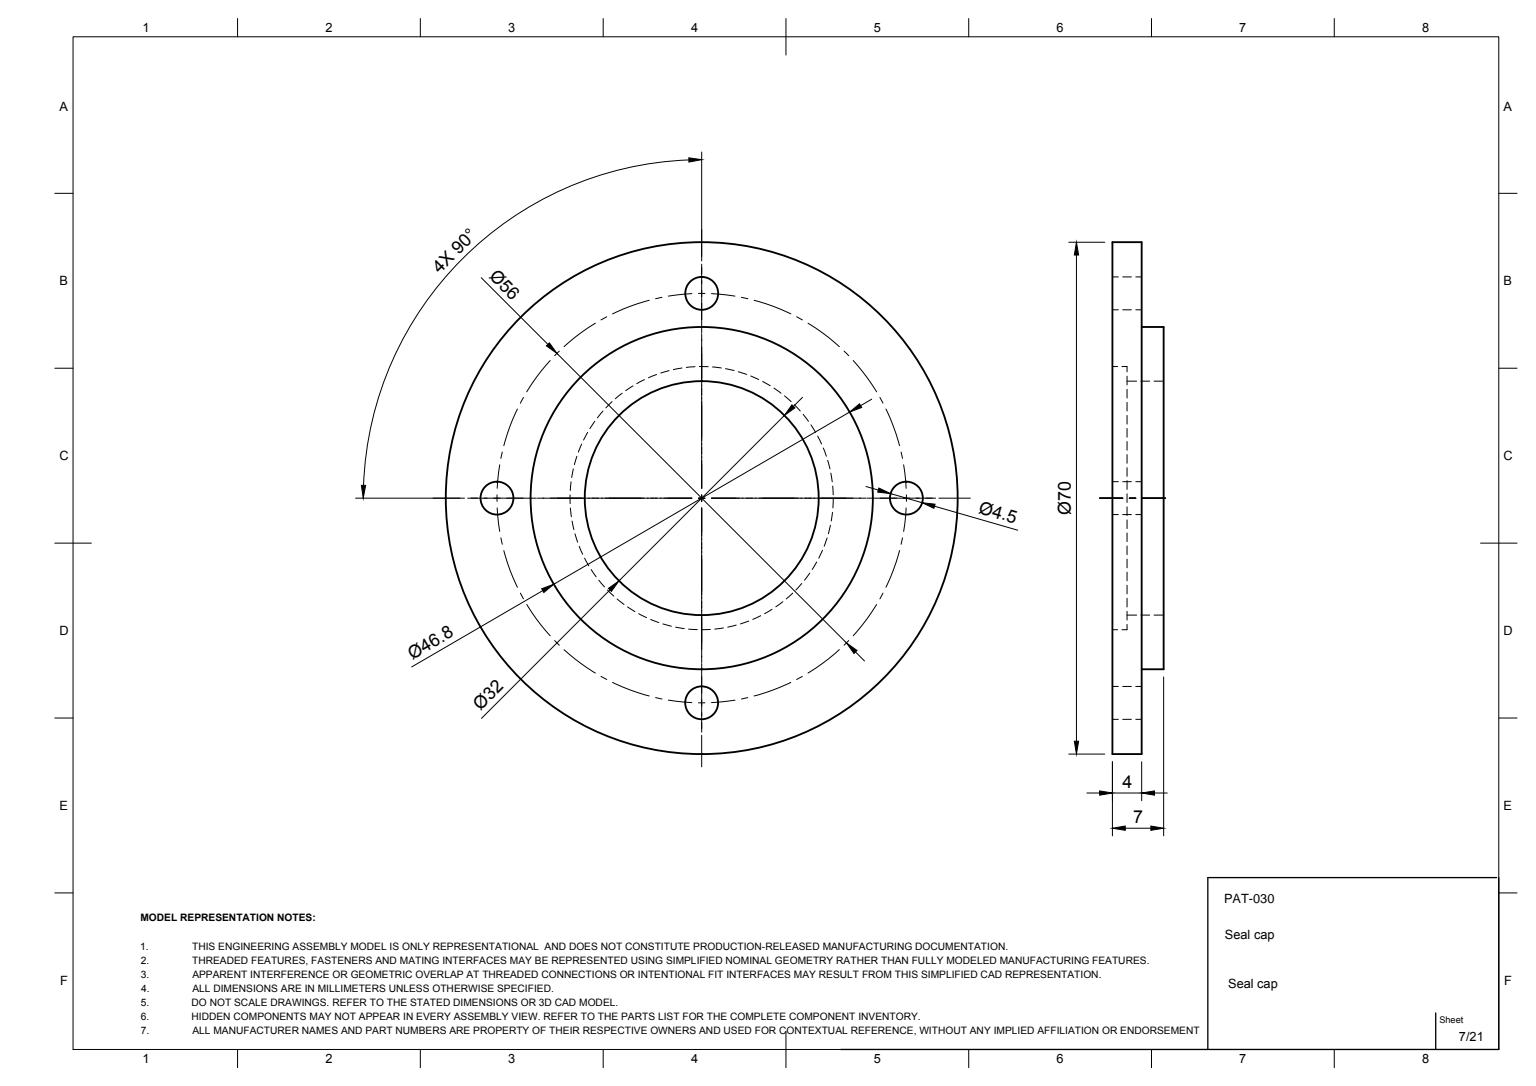
ISO-10303-21;
HEADER;
/* Generated by software containing ST-Developer
 * from STEP Tools, Inc. (www.steptools.com) 
 */

FILE_DESCRIPTION(
/* description */ ('Double-bearing flanged cartridge'),
/* implementation_level */ '2;1');

FILE_NAME(
/* name */ 'Seal cap.step',
/* time_stamp */ '2026-10-28T03:26:40-07:00',
/* author */ (''),
/* organization */ (''),
/* preprocessor_version */ 'ST-DEVELOPER v20.2',
/* originating_system */ 'Autodesk Translation Framework v15.17.0.0',
/* authorisation */ '');

FILE_SCHEMA (('AUTOMOTIVE_DESIGN { 1 0 10303 214 3 1 1 }'));
ENDSEC;

DATA;
#10=MECHANICAL_DESIGN_GEOMETRIC_PRESENTATION_REPRESENTATION('',(#205),#5535);
#169=SHAPE_REPRESENTATION_RELATIONSHIP('SRR','None',#5611,#183);
#183=ADVANCED_BREP_SHAPE_REPRESENTATION('',(#227),#5527);
#205=STYLED_ITEM('',(#5771),#227);
#227=MANIFOLD_SOLID_BREP('Body1',#2339);
#264=FACE_BOUND('',#630,.T.);
#265=FACE_BOUND('',#633,.T.);
#266=FACE_BOUND('',#637,.T.);
#267=FACE_BOUND('',#638,.T.);
#268=FACE_BOUND('',#639,.T.);
#269=FACE_BOUND('',#640,.T.);
#270=FACE_BOUND('',#641,.T.);
#271=FACE_BOUND('',#643,.T.);
#272=FACE_BOUND('',#644,.T.);
#273=FACE_BOUND('',#645,.T.);
#274=FACE_BOUND('',#646,.T.);
#275=FACE_BOUND('',#647,.T.);
#331=PLANE('',#2724);
#332=PLANE('',#2729);
#333=PLANE('',#2735);
#334=PLANE('',#2736);
#444=FACE_OUTER_BOUND('',#624,.T.);
#445=FACE_OUTER_BOUND('',#625,.T.);
#446=FACE_OUTER_BOUND('',#626,.T.);
#447=FACE_OUTER_BOUND('',#627,.T.);
#448=FACE_OUTER_BOUND('',#628,.T.);
#449=FACE_OUTER_BOUND('',#629,.T.);
#450=FACE_OUTER_BOUND('',#631,.T.);
#451=FACE_OUTER_BOUND('',#632,.T.);
#452=FACE_OUTER_BOUND('',#634,.T.);
#453=FACE_OUTER_BOUND('',#635,.T.);
#454=FACE_OUTER_BOUND('',#636,.T.);
#455=FACE_OUTER_BOUND('',#642,.T.);
#624=EDGE_LOOP('',(#1870,#1871,#1872,#1873));
#625=EDGE_LOOP('',(#1874,#1875,#1876,#1877));
#626=EDGE_LOOP('',(#1878,#1879,#1880,#1881));
#627=EDGE_LOOP('',(#1882,#1883,#1884,#1885));
#628=EDGE_LOOP('',(#1886,#1887,#1888,#1889));
#629=EDGE_LOOP('',(#1890));
#630=EDGE_LOOP('',(#1891));
#631=EDGE_LOOP('',(#1892,#1893,#1894,#1895));
#632=EDGE_LOOP('',(#1896));
#633=EDGE_LOOP('',(#1897));
#634=EDGE_LOOP('',(#1898,#1899,#1900,#1901));
#635=EDGE_LOOP('',(#1902,#1903,#1904,#1905));
#636=EDGE_LOOP('',(#1906));
#637=EDGE_LOOP('',(#1907));
#638=EDGE_LOOP('',(#1908));
#639=EDGE_LOOP('',(#1909));
#640=EDGE_LOOP('',(#1910));
#641=EDGE_LOOP('',(#1911));
#642=EDGE_LOOP('',(#1912));
#643=EDGE_LOOP('',(#1913));
#644=EDGE_LOOP('',(#1914));
#645=EDGE_LOOP('',(#1915));
#646=EDGE_LOOP('',(#1916));
#647=EDGE_LOOP('',(#1917));
#760=LINE('',#4400,#846);
#761=LINE('',#4406,#847);
#762=LINE('',#4412,#848);
#763=LINE('',#4418,#849);
#764=LINE('',#4424,#850);
#765=LINE('',#4433,#851);
#766=LINE('',#4439,#852);
#767=LINE('',#4444,#853);
#846=VECTOR('',#3319,0.225);
#847=VECTOR('',#3326,0.225);
#848=VECTOR('',#3333,0.225);
#849=VECTOR('',#3340,0.225);
#850=VECTOR('',#3347,2.34);
#851=VECTOR('',#3358,1.8);
#852=VECTOR('',#3367,1.6);
#853=VECTOR('',#3372,3.5);
#1006=CIRCLE('',#2710,0.225);
#1007=CIRCLE('',#2711,0.225);
#1008=CIRCLE('',#2713,0.225);
#1009=CIRCLE('',#2714,0.225);
#1010=CIRCLE('',#2716,0.225);
#1011=CIRCLE('',#2717,0.225);
#1012=CIRCLE('',#2719,0.225);
#1013=CIRCLE('',#2720,0.225);
#1014=CIRCLE('',#2722,2.34);
#1015=CIRCLE('',#2723,2.34);
#1016=CIRCLE('',#2725,1.6);
#1017=CIRCLE('',#2727,1.8);
#1018=CIRCLE('',#2728,1.8);
#1019=CIRCLE('',#2730,1.6);
#1020=CIRCLE('',#2733,3.5);
#1021=CIRCLE('',#2734,3.5);
#1188=VERTEX_POINT('',#4397);
#1189=VERTEX_POINT('',#4399);
#1190=VERTEX_POINT('',#4403);
#1191=VERTEX_POINT('',#4405);
#1192=VERTEX_POINT('',#4409);
#1193=VERTEX_POINT('',#4411);
#1194=VERTEX_POINT('',#4415);
#1195=VERTEX_POINT('',#4417);
#1196=VERTEX_POINT('',#4421);
#1197=VERTEX_POINT('',#4423);
#1198=VERTEX_POINT('',#4427);
#1199=VERTEX_POINT('',#4430);
#1200=VERTEX_POINT('',#4432);
#1201=VERTEX_POINT('',#4436);
#1202=VERTEX_POINT('',#4441);
#1203=VERTEX_POINT('',#4443);
#1428=EDGE_CURVE('',#1188,#1188,#1006,.T.);
#1429=EDGE_CURVE('',#1188,#1189,#760,.T.);
#1430=EDGE_CURVE('',#1189,#1189,#1007,.T.);
#1431=EDGE_CURVE('',#1190,#1190,#1008,.T.);
#1432=EDGE_CURVE('',#1190,#1191,#761,.T.);
#1433=EDGE_CURVE('',#1191,#1191,#1009,.T.);
#1434=EDGE_CURVE('',#1192,#1192,#1010,.T.);
#1435=EDGE_CURVE('',#1192,#1193,#762,.T.);
#1436=EDGE_CURVE('',#1193,#1193,#1011,.T.);
#1437=EDGE_CURVE('',#1194,#1194,#1012,.T.);
#1438=EDGE_CURVE('',#1194,#1195,#763,.T.);
#1439=EDGE_CURVE('',#1195,#1195,#1013,.T.);
#1440=EDGE_CURVE('',#1196,#1196,#1014,.T.);
#1441=EDGE_CURVE('',#1196,#1197,#764,.T.);
#1442=EDGE_CURVE('',#1197,#1197,#1015,.T.);
#1443=EDGE_CURVE('',#1198,#1198,#1016,.T.);
#1444=EDGE_CURVE('',#1199,#1199,#1017,.T.);
#1445=EDGE_CURVE('',#1199,#1200,#765,.T.);
#1446=EDGE_CURVE('',#1200,#1200,#1018,.T.);
#1447=EDGE_CURVE('',#1201,#1201,#1019,.T.);
#1448=EDGE_CURVE('',#1198,#1201,#766,.T.);
#1449=EDGE_CURVE('',#1202,#1202,#1020,.T.);
#1450=EDGE_CURVE('',#1202,#1203,#767,.T.);
#1451=EDGE_CURVE('',#1203,#1203,#1021,.T.);
#1870=ORIENTED_EDGE('',*,*,#1428,.F.);
#1871=ORIENTED_EDGE('',*,*,#1429,.T.);
#1872=ORIENTED_EDGE('',*,*,#1430,.F.);
#1873=ORIENTED_EDGE('',*,*,#1429,.F.);
#1874=ORIENTED_EDGE('',*,*,#1431,.F.);
#1875=ORIENTED_EDGE('',*,*,#1432,.T.);
#1876=ORIENTED_EDGE('',*,*,#1433,.F.);
#1877=ORIENTED_EDGE('',*,*,#1432,.F.);
#1878=ORIENTED_EDGE('',*,*,#1434,.F.);
#1879=ORIENTED_EDGE('',*,*,#1435,.T.);
#1880=ORIENTED_EDGE('',*,*,#1436,.F.);
#1881=ORIENTED_EDGE('',*,*,#1435,.F.);
#1882=ORIENTED_EDGE('',*,*,#1437,.F.);
#1883=ORIENTED_EDGE('',*,*,#1438,.T.);
#1884=ORIENTED_EDGE('',*,*,#1439,.F.);
#1885=ORIENTED_EDGE('',*,*,#1438,.F.);
#1886=ORIENTED_EDGE('',*,*,#1440,.F.);
#1887=ORIENTED_EDGE('',*,*,#1441,.T.);
#1888=ORIENTED_EDGE('',*,*,#1442,.F.);
#1889=ORIENTED_EDGE('',*,*,#1441,.F.);
#1890=ORIENTED_EDGE('',*,*,#1440,.T.);
#1891=ORIENTED_EDGE('',*,*,#1443,.T.);
#1892=ORIENTED_EDGE('',*,*,#1444,.F.);
#1893=ORIENTED_EDGE('',*,*,#1445,.T.);
#1894=ORIENTED_EDGE('',*,*,#1446,.T.);
#1895=ORIENTED_EDGE('',*,*,#1445,.F.);
#1896=ORIENTED_EDGE('',*,*,#1446,.F.);
#1897=ORIENTED_EDGE('',*,*,#1447,.F.);
#1898=ORIENTED_EDGE('',*,*,#1443,.F.);
#1899=ORIENTED_EDGE('',*,*,#1448,.T.);
#1900=ORIENTED_EDGE('',*,*,#1447,.T.);
#1901=ORIENTED_EDGE('',*,*,#1448,.F.);
#1902=ORIENTED_EDGE('',*,*,#1449,.F.);
#1903=ORIENTED_EDGE('',*,*,#1450,.T.);
#1904=ORIENTED_EDGE('',*,*,#1451,.T.);
#1905=ORIENTED_EDGE('',*,*,#1450,.F.);
#1906=ORIENTED_EDGE('',*,*,#1449,.T.);
#1907=ORIENTED_EDGE('',*,*,#1442,.T.);
#1908=ORIENTED_EDGE('',*,*,#1439,.T.);
#1909=ORIENTED_EDGE('',*,*,#1436,.T.);
#1910=ORIENTED_EDGE('',*,*,#1433,.T.);
#1911=ORIENTED_EDGE('',*,*,#1430,.T.);
#1912=ORIENTED_EDGE('',*,*,#1451,.F.);
#1913=ORIENTED_EDGE('',*,*,#1444,.T.);
#1914=ORIENTED_EDGE('',*,*,#1437,.T.);
#1915=ORIENTED_EDGE('',*,*,#1434,.T.);
#1916=ORIENTED_EDGE('',*,*,#1431,.T.);
#1917=ORIENTED_EDGE('',*,*,#1428,.T.);
#2144=CYLINDRICAL_SURFACE('',#2709,0.225);
#2145=CYLINDRICAL_SURFACE('',#2712,0.225);
#2146=CYLINDRICAL_SURFACE('',#2715,0.225);
#2147=CYLINDRICAL_SURFACE('',#2718,0.225);
#2148=CYLINDRICAL_SURFACE('',#2721,2.34);
#2149=CYLINDRICAL_SURFACE('',#2726,1.8);
#2150=CYLINDRICAL_SURFACE('',#2731,1.6);
#2151=CYLINDRICAL_SURFACE('',#2732,3.5);
#2258=ADVANCED_FACE('',(#444),#2144,.F.);
#2259=ADVANCED_FACE('',(#445),#2145,.F.);
#2260=ADVANCED_FACE('',(#446),#2146,.F.);
#2261=ADVANCED_FACE('',(#447),#2147,.F.);
#2262=ADVANCED_FACE('',(#448),#2148,.T.);
#2263=ADVANCED_FACE('',(#449,#264),#331,.T.);
#2264=ADVANCED_FACE('',(#450),#2149,.F.);
#2265=ADVANCED_FACE('',(#451,#265),#332,.F.);
#2266=ADVANCED_FACE('',(#452),#2150,.F.);
#2267=ADVANCED_FACE('',(#453),#2151,.T.);
#2268=ADVANCED_FACE('',(#454,#266,#267,#268,#269,#270),#333,.T.);
#2269=ADVANCED_FACE('',(#455,#271,#272,#273,#274,#275),#334,.F.);
#2339=CLOSED_SHELL('',(#2258,#2259,#2260,#2261,#2262,#2263,#2264,#2265,
#2266,#2267,#2268,#2269));
#2708=AXIS2_PLACEMENT_3D('',#4395,#3313,#3314);
#2709=AXIS2_PLACEMENT_3D('',#4396,#3315,#3316);
#2710=AXIS2_PLACEMENT_3D('',#4398,#3317,#3318);
#2711=AXIS2_PLACEMENT_3D('',#4401,#3320,#3321);
#2712=AXIS2_PLACEMENT_3D('',#4402,#3322,#3323);
#2713=AXIS2_PLACEMENT_3D('',#4404,#3324,#3325);
#2714=AXIS2_PLACEMENT_3D('',#4407,#3327,#3328);
#2715=AXIS2_PLACEMENT_3D('',#4408,#3329,#3330);
#2716=AXIS2_PLACEMENT_3D('',#4410,#3331,#3332);
#2717=AXIS2_PLACEMENT_3D('',#4413,#3334,#3335);
#2718=AXIS2_PLACEMENT_3D('',#4414,#3336,#3337);
#2719=AXIS2_PLACEMENT_3D('',#4416,#3338,#3339);
#2720=AXIS2_PLACEMENT_3D('',#4419,#3341,#3342);
#2721=AXIS2_PLACEMENT_3D('',#4420,#3343,#3344);
#2722=AXIS2_PLACEMENT_3D('',#4422,#3345,#3346);
#2723=AXIS2_PLACEMENT_3D('',#4425,#3348,#3349);
#2724=AXIS2_PLACEMENT_3D('',#4426,#3350,#3351);
#2725=AXIS2_PLACEMENT_3D('',#4428,#3352,#3353);
#2726=AXIS2_PLACEMENT_3D('',#4429,#3354,#3355);
#2727=AXIS2_PLACEMENT_3D('',#4431,#3356,#3357);
#2728=AXIS2_PLACEMENT_3D('',#4434,#3359,#3360);
#2729=AXIS2_PLACEMENT_3D('',#4435,#3361,#3362);
#2730=AXIS2_PLACEMENT_3D('',#4437,#3363,#3364);
#2731=AXIS2_PLACEMENT_3D('',#4438,#3365,#3366);
#2732=AXIS2_PLACEMENT_3D('',#4440,#3368,#3369);
#2733=AXIS2_PLACEMENT_3D('',#4442,#3370,#3371);
#2734=AXIS2_PLACEMENT_3D('',#4445,#3373,#3374);
#2735=AXIS2_PLACEMENT_3D('',#4446,#3375,#3376);
#2736=AXIS2_PLACEMENT_3D('',#4447,#3377,#3378);
#3313=DIRECTION('axis',(0.,0.,1.));
#3314=DIRECTION('refdir',(1.,0.,0.));
#3315=DIRECTION('center_axis',(0.,1.,0.));
#3316=DIRECTION('ref_axis',(1.,0.,0.));
#3317=DIRECTION('center_axis',(0.,1.,0.));
#3318=DIRECTION('ref_axis',(1.,0.,0.));
#3319=DIRECTION('',(0.,1.,0.));
#3320=DIRECTION('center_axis',(0.,-1.,0.));
#3321=DIRECTION('ref_axis',(1.,0.,0.));
#3322=DIRECTION('center_axis',(0.,1.,0.));
#3323=DIRECTION('ref_axis',(1.,0.,0.));
#3324=DIRECTION('center_axis',(0.,1.,0.));
#3325=DIRECTION('ref_axis',(1.,0.,0.));
#3326=DIRECTION('',(0.,1.,0.));
#3327=DIRECTION('center_axis',(0.,-1.,0.));
#3328=DIRECTION('ref_axis',(1.,0.,0.));
#3329=DIRECTION('center_axis',(0.,1.,0.));
#3330=DIRECTION('ref_axis',(1.,0.,0.));
#3331=DIRECTION('center_axis',(0.,1.,0.));
#3332=DIRECTION('ref_axis',(1.,0.,0.));
#3333=DIRECTION('',(0.,1.,0.));
#3334=DIRECTION('center_axis',(0.,-1.,0.));
#3335=DIRECTION('ref_axis',(1.,0.,0.));
#3336=DIRECTION('center_axis',(0.,1.,0.));
#3337=DIRECTION('ref_axis',(1.,0.,0.));
#3338=DIRECTION('center_axis',(0.,1.,0.));
#3339=DIRECTION('ref_axis',(1.,0.,0.));
#3340=DIRECTION('',(0.,1.,0.));
#3341=DIRECTION('center_axis',(0.,-1.,0.));
#3342=DIRECTION('ref_axis',(1.,0.,0.));
#3343=DIRECTION('center_axis',(0.,1.,0.));
#3344=DIRECTION('ref_axis',(1.,0.,0.));
#3345=DIRECTION('center_axis',(0.,1.,0.));
#3346=DIRECTION('ref_axis',(1.,0.,0.));
#3347=DIRECTION('',(0.,-1.,0.));
#3348=DIRECTION('center_axis',(0.,-1.,0.));
#3349=DIRECTION('ref_axis',(1.,0.,0.));
#3350=DIRECTION('center_axis',(0.,1.,0.));
#3351=DIRECTION('ref_axis',(1.,0.,0.));
#3352=DIRECTION('center_axis',(0.,-1.,0.));
#3353=DIRECTION('ref_axis',(1.,0.,0.));
#3354=DIRECTION('center_axis',(0.,1.,0.));
#3355=DIRECTION('ref_axis',(1.,0.,0.));
#3356=DIRECTION('center_axis',(0.,1.,0.));
#3357=DIRECTION('ref_axis',(1.,0.,0.));
#3358=DIRECTION('',(0.,1.,0.));
#3359=DIRECTION('center_axis',(0.,1.,0.));
#3360=DIRECTION('ref_axis',(1.,0.,0.));
#3361=DIRECTION('center_axis',(0.,1.,0.));
#3362=DIRECTION('ref_axis',(1.,0.,0.));
#3363=DIRECTION('center_axis',(0.,-1.,0.));
#3364=DIRECTION('ref_axis',(1.,0.,0.));
#3365=DIRECTION('center_axis',(0.,1.,0.));
#3366=DIRECTION('ref_axis',(1.,0.,0.));
#3367=DIRECTION('',(0.,-1.,0.));
#3368=DIRECTION('center_axis',(0.,1.,0.));
#3369=DIRECTION('ref_axis',(1.,0.,0.));
#3370=DIRECTION('center_axis',(0.,1.,0.));
#3371=DIRECTION('ref_axis',(1.,0.,0.));
#3372=DIRECTION('',(0.,-1.,0.));
#3373=DIRECTION('center_axis',(0.,1.,0.));
#3374=DIRECTION('ref_axis',(1.,0.,0.));
#3375=DIRECTION('center_axis',(0.,1.,0.));
#3376=DIRECTION('ref_axis',(1.,0.,0.));
#3377=DIRECTION('center_axis',(0.,1.,0.));
#3378=DIRECTION('ref_axis',(1.,0.,0.));
#4395=CARTESIAN_POINT('',(0.,0.,0.));
#4396=CARTESIAN_POINT('Origin',(-2.8,-0.5,4.5));
#4397=CARTESIAN_POINT('',(-3.025,-0.4,4.5));
#4398=CARTESIAN_POINT('Origin',(-2.8,-0.4,4.5));
#4399=CARTESIAN_POINT('',(-3.025,0.,4.5));
#4400=CARTESIAN_POINT('',(-3.025,-0.5,4.5));
#4401=CARTESIAN_POINT('Origin',(-2.8,0.,4.5));
#4402=CARTESIAN_POINT('Origin',(1.71450551880629E-16,-0.5,7.3));
#4403=CARTESIAN_POINT('',(-0.225,-0.4,7.3));
#4404=CARTESIAN_POINT('Origin',(1.71450551880629E-16,-0.4,7.3));
#4405=CARTESIAN_POINT('',(-0.225,0.,7.3));
#4406=CARTESIAN_POINT('',(-0.225,-0.5,7.3));
#4407=CARTESIAN_POINT('Origin',(1.71450551880629E-16,0.,7.3));
#4408=CARTESIAN_POINT('Origin',(2.8,-0.5,4.5));
#4409=CARTESIAN_POINT('',(2.575,-0.4,4.5));
#4410=CARTESIAN_POINT('Origin',(2.8,-0.4,4.5));
#4411=CARTESIAN_POINT('',(2.575,0.,4.5));
#4412=CARTESIAN_POINT('',(2.575,-0.5,4.5));
#4413=CARTESIAN_POINT('Origin',(2.8,0.,4.5));
#4414=CARTESIAN_POINT('Origin',(-5.14351655641888E-16,-0.5,1.7));
#4415=CARTESIAN_POINT('',(-0.225000000000001,-0.4,1.7));
#4416=CARTESIAN_POINT('Origin',(-5.14351655641888E-16,-0.4,1.7));
#4417=CARTESIAN_POINT('',(-0.225000000000001,0.,1.7));
#4418=CARTESIAN_POINT('',(-0.225000000000001,-0.5,1.7));
#4419=CARTESIAN_POINT('Origin',(-5.14351655641888E-16,0.,1.7));
#4420=CARTESIAN_POINT('Origin',(0.,0.,4.5));
#4421=CARTESIAN_POINT('',(-2.34,0.3,4.5));
#4422=CARTESIAN_POINT('Origin',(0.,0.3,4.5));
#4423=CARTESIAN_POINT('',(-2.34,0.,4.5));
#4424=CARTESIAN_POINT('',(-2.34,0.,4.5));
#4425=CARTESIAN_POINT('Origin',(0.,0.,4.5));
#4426=CARTESIAN_POINT('Origin',(0.,0.3,4.5));
#4427=CARTESIAN_POINT('',(-1.6,0.3,4.5));
#4428=CARTESIAN_POINT('Origin',(0.,0.3,4.5));
#4429=CARTESIAN_POINT('Origin',(0.,-0.41,4.5));
#4430=CARTESIAN_POINT('',(-1.8,-0.4,4.5));
#4431=CARTESIAN_POINT('Origin',(0.,-0.4,4.5));
#4432=CARTESIAN_POINT('',(-1.8,-0.2,4.5));
#4433=CARTESIAN_POINT('',(-1.8,-0.41,4.5));
#4434=CARTESIAN_POINT('Origin',(0.,-0.2,4.5));
#4435=CARTESIAN_POINT('Origin',(0.,-0.2,4.5));
#4436=CARTESIAN_POINT('',(-1.6,-0.2,4.5));
#4437=CARTESIAN_POINT('Origin',(0.,-0.2,4.5));
#4438=CARTESIAN_POINT('Origin',(0.,-0.4,4.5));
#4439=CARTESIAN_POINT('',(-1.6,-0.4,4.5));
#4440=CARTESIAN_POINT('Origin',(0.,-0.4,4.5));
#4441=CARTESIAN_POINT('',(-3.5,0.,4.5));
#4442=CARTESIAN_POINT('Origin',(0.,0.,4.5));
#4443=CARTESIAN_POINT('',(-3.5,-0.4,4.5));
#4444=CARTESIAN_POINT('',(-3.5,-0.4,4.5));
#4445=CARTESIAN_POINT('Origin',(0.,-0.4,4.5));
#4446=CARTESIAN_POINT('Origin',(0.,0.,4.5));
#4447=CARTESIAN_POINT('Origin',(0.,-0.4,4.5));
#5508=UNCERTAINTY_MEASURE_WITH_UNIT(LENGTH_MEASURE(0.001),#5536,
'DISTANCE_ACCURACY_VALUE',
'Maximum model space distance between geometric entities at asserted c
onnectivities');
#5516=UNCERTAINTY_MEASURE_WITH_UNIT(LENGTH_MEASURE(0.001),#5536,
'DISTANCE_ACCURACY_VALUE',
'Maximum model space distance between geometric entities at asserted c
onnectivities');
#5527=(
GEOMETRIC_REPRESENTATION_CONTEXT(3)
GLOBAL_UNCERTAINTY_ASSIGNED_CONTEXT((#5508))
GLOBAL_UNIT_ASSIGNED_CONTEXT((#5536,#5538,#5539))
REPRESENTATION_CONTEXT('','3D')
);
#5535=(
GEOMETRIC_REPRESENTATION_CONTEXT(3)
GLOBAL_UNCERTAINTY_ASSIGNED_CONTEXT((#5516))
GLOBAL_UNIT_ASSIGNED_CONTEXT((#5536,#5538,#5539))
REPRESENTATION_CONTEXT('','3D')
);
#5536=(
LENGTH_UNIT()
NAMED_UNIT(*)
SI_UNIT(.CENTI.,.METRE.)
);
#5538=(
NAMED_UNIT(*)
PLANE_ANGLE_UNIT()
SI_UNIT($,.RADIAN.)
);
#5539=(
NAMED_UNIT(*)
SI_UNIT($,.STERADIAN.)
SOLID_ANGLE_UNIT()
);
#5550=SHAPE_DEFINITION_REPRESENTATION(#5573,#5611);
#5573=PRODUCT_DEFINITION_SHAPE('',$,#5630);
#5611=SHAPE_REPRESENTATION('',(#2708),#5527);
#5619=PRODUCT_DEFINITION_CONTEXT('part definition',#5675,'design');
#5630=PRODUCT_DEFINITION('Seal cap','Seal cap',#5648,#5619);
#5648=PRODUCT_DEFINITION_FORMATION('',$,#5687);
#5675=APPLICATION_CONTEXT(
'Core Data for Automotive Mechanical Design Process');
#5676=PRODUCT_CONTEXT('part definition',#5675,'mechanical');
#5687=PRODUCT('Seal cap','Seal cap','Seal cap',(#5676));
#5765=COLOUR_RGB('Black',0.12,0.14,0.17);
#5766=FILL_AREA_STYLE_COLOUR('',#5765);
#5767=FILL_AREA_STYLE('',(#5766));
#5768=SURFACE_STYLE_FILL_AREA(#5767);
#5769=SURFACE_SIDE_STYLE('',(#5768));
#5770=SURFACE_STYLE_USAGE(.BOTH.,#5769);
#5771=PRESENTATION_STYLE_ASSIGNMENT((#5770));
ENDSEC;
END-ISO-10303-21;
